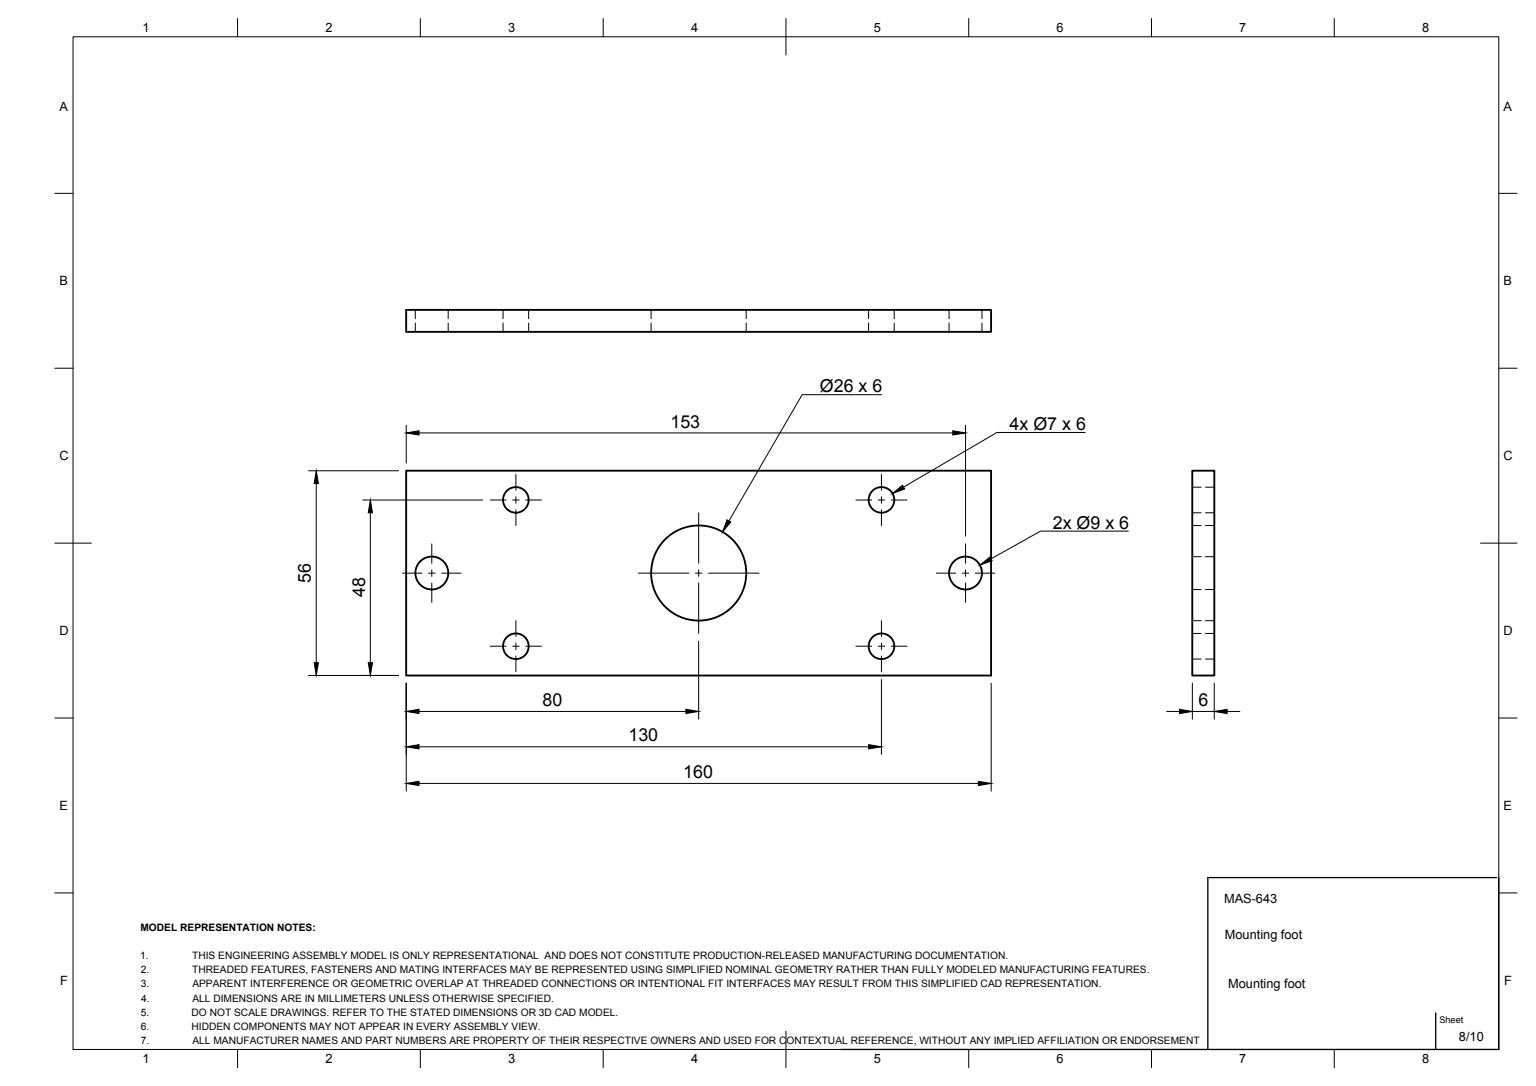
ISO-10303-21;
HEADER;
/* Generated by software containing ST-Developer
 * from STEP Tools, Inc. (www.steptools.com) 
 */

FILE_DESCRIPTION(
/* description */ ('Independent eighteen-tube parallel-flow evaporator geometry. Repeated
 machined headers and gasketed service covers, eighteen copper tubes, 
twenty-nine punched fins, threaded hose connections and bolted mountin
g feet. Native editable features and instanced parts. Braze details, w
orking fluid, pressure and thermal ratings require engineering selecti
on.'),
/* implementation_level */ '2;1');

FILE_NAME(
/* name */ 'Mounting foot.step',
/* time_stamp */ '2026-11-08T20:53:59-08:00',
/* author */ (''),
/* organization */ (''),
/* preprocessor_version */ 'ST-DEVELOPER v20.2',
/* originating_system */ 'Autodesk Translation Framework v15.17.0.0',
/* authorisation */ '');

FILE_SCHEMA (('AUTOMOTIVE_DESIGN { 1 0 10303 214 3 1 1 }'));
ENDSEC;

DATA;
#10=MECHANICAL_DESIGN_GEOMETRIC_PRESENTATION_REPRESENTATION('',(#338),#42620);
#318=SHAPE_REPRESENTATION_RELATIONSHIP('SRR','None',#42728,#328);
#328=ADVANCED_BREP_SHAPE_REPRESENTATION('',(#348),#42615);
#338=STYLED_ITEM('',(#42787),#348);
#348=MANIFOLD_SOLID_BREP('Body1',#10388);
#457=FACE_BOUND('',#1662,.T.);
#458=FACE_BOUND('',#1663,.T.);
#459=FACE_BOUND('',#1664,.T.);
#460=FACE_BOUND('',#1665,.T.);
#461=FACE_BOUND('',#1666,.T.);
#462=FACE_BOUND('',#1667,.T.);
#463=FACE_BOUND('',#1668,.T.);
#464=FACE_BOUND('',#1670,.T.);
#465=FACE_BOUND('',#1671,.T.);
#466=FACE_BOUND('',#1672,.T.);
#467=FACE_BOUND('',#1673,.T.);
#468=FACE_BOUND('',#1674,.T.);
#469=FACE_BOUND('',#1675,.T.);
#470=FACE_BOUND('',#1676,.T.);
#541=PLANE('',#11055);
#542=PLANE('',#11056);
#543=PLANE('',#11057);
#544=PLANE('',#11058);
#545=PLANE('',#11059);
#546=PLANE('',#11060);
#1002=FACE_OUTER_BOUND('',#1650,.T.);
#1003=FACE_OUTER_BOUND('',#1651,.T.);
#1004=FACE_OUTER_BOUND('',#1652,.T.);
#1005=FACE_OUTER_BOUND('',#1653,.T.);
#1006=FACE_OUTER_BOUND('',#1654,.T.);
#1007=FACE_OUTER_BOUND('',#1655,.T.);
#1008=FACE_OUTER_BOUND('',#1656,.T.);
#1009=FACE_OUTER_BOUND('',#1657,.T.);
#1010=FACE_OUTER_BOUND('',#1658,.T.);
#1011=FACE_OUTER_BOUND('',#1659,.T.);
#1012=FACE_OUTER_BOUND('',#1660,.T.);
#1013=FACE_OUTER_BOUND('',#1661,.T.);
#1014=FACE_OUTER_BOUND('',#1669,.T.);
#1650=EDGE_LOOP('',(#8675,#8676,#8677,#8678));
#1651=EDGE_LOOP('',(#8679,#8680,#8681,#8682));
#1652=EDGE_LOOP('',(#8683,#8684,#8685,#8686));
#1653=EDGE_LOOP('',(#8687,#8688,#8689,#8690));
#1654=EDGE_LOOP('',(#8691,#8692,#8693,#8694));
#1655=EDGE_LOOP('',(#8695,#8696,#8697,#8698));
#1656=EDGE_LOOP('',(#8699,#8700,#8701,#8702));
#1657=EDGE_LOOP('',(#8703,#8704,#8705,#8706));
#1658=EDGE_LOOP('',(#8707,#8708,#8709,#8710));
#1659=EDGE_LOOP('',(#8711,#8712,#8713,#8714));
#1660=EDGE_LOOP('',(#8715,#8716,#8717,#8718));
#1661=EDGE_LOOP('',(#8719,#8720,#8721,#8722));
#1662=EDGE_LOOP('',(#8723));
#1663=EDGE_LOOP('',(#8724));
#1664=EDGE_LOOP('',(#8725));
#1665=EDGE_LOOP('',(#8726));
#1666=EDGE_LOOP('',(#8727));
#1667=EDGE_LOOP('',(#8728));
#1668=EDGE_LOOP('',(#8729));
#1669=EDGE_LOOP('',(#8730,#8731,#8732,#8733));
#1670=EDGE_LOOP('',(#8734));
#1671=EDGE_LOOP('',(#8735));
#1672=EDGE_LOOP('',(#8736));
#1673=EDGE_LOOP('',(#8737));
#1674=EDGE_LOOP('',(#8738));
#1675=EDGE_LOOP('',(#8739));
#1676=EDGE_LOOP('',(#8740));
#1967=CIRCLE('',#11035,13.);
#1968=CIRCLE('',#11036,13.);
#1969=CIRCLE('',#11038,4.5);
#1970=CIRCLE('',#11039,4.5);
#1971=CIRCLE('',#11041,4.5);
#1972=CIRCLE('',#11042,4.5);
#1973=CIRCLE('',#11044,3.5);
#1974=CIRCLE('',#11045,3.5);
#1975=CIRCLE('',#11047,3.5);
#1976=CIRCLE('',#11048,3.5);
#1977=CIRCLE('',#11050,3.5);
#1978=CIRCLE('',#11051,3.5);
#1979=CIRCLE('',#11053,3.5);
#1980=CIRCLE('',#11054,3.5);
#3194=LINE('',#35119,#3732);
#3195=LINE('',#35125,#3733);
#3196=LINE('',#35131,#3734);
#3197=LINE('',#35137,#3735);
#3198=LINE('',#35143,#3736);
#3199=LINE('',#35149,#3737);
#3200=LINE('',#35155,#3738);
#3201=LINE('',#35160,#3739);
#3202=LINE('',#35162,#3740);
#3203=LINE('',#35164,#3741);
#3204=LINE('',#35165,#3742);
#3205=LINE('',#35168,#3743);
#3206=LINE('',#35170,#3744);
#3207=LINE('',#35171,#3745);
#3208=LINE('',#35174,#3746);
#3209=LINE('',#35176,#3747);
#3210=LINE('',#35177,#3748);
#3211=LINE('',#35179,#3749);
#3212=LINE('',#35180,#3750);
#3732=VECTOR('',#12765,13.);
#3733=VECTOR('',#12772,4.5);
#3734=VECTOR('',#12779,4.5);
#3735=VECTOR('',#12786,3.5);
#3736=VECTOR('',#12793,3.5);
#3737=VECTOR('',#12800,3.5);
#3738=VECTOR('',#12807,3.5);
#3739=VECTOR('',#12812,10.);
#3740=VECTOR('',#12813,10.);
#3741=VECTOR('',#12814,10.);
#3742=VECTOR('',#12815,10.);
#3743=VECTOR('',#12818,10.);
#3744=VECTOR('',#12819,10.);
#3745=VECTOR('',#12820,10.);
#3746=VECTOR('',#12823,10.);
#3747=VECTOR('',#12824,10.);
#3748=VECTOR('',#12825,10.);
#3749=VECTOR('',#12828,10.);
#3750=VECTOR('',#12829,10.);
#4631=VERTEX_POINT('',#35116);
#4632=VERTEX_POINT('',#35118);
#4633=VERTEX_POINT('',#35122);
#4634=VERTEX_POINT('',#35124);
#4635=VERTEX_POINT('',#35128);
#4636=VERTEX_POINT('',#35130);
#4637=VERTEX_POINT('',#35134);
#4638=VERTEX_POINT('',#35136);
#4639=VERTEX_POINT('',#35140);
#4640=VERTEX_POINT('',#35142);
#4641=VERTEX_POINT('',#35146);
#4642=VERTEX_POINT('',#35148);
#4643=VERTEX_POINT('',#35152);
#4644=VERTEX_POINT('',#35154);
#4645=VERTEX_POINT('',#35158);
#4646=VERTEX_POINT('',#35159);
#4647=VERTEX_POINT('',#35161);
#4648=VERTEX_POINT('',#35163);
#4649=VERTEX_POINT('',#35167);
#4650=VERTEX_POINT('',#35169);
#4651=VERTEX_POINT('',#35173);
#4652=VERTEX_POINT('',#35175);
#6020=EDGE_CURVE('',#4631,#4631,#1967,.T.);
#6021=EDGE_CURVE('',#4631,#4632,#3194,.T.);
#6022=EDGE_CURVE('',#4632,#4632,#1968,.T.);
#6023=EDGE_CURVE('',#4633,#4633,#1969,.T.);
#6024=EDGE_CURVE('',#4633,#4634,#3195,.T.);
#6025=EDGE_CURVE('',#4634,#4634,#1970,.T.);
#6026=EDGE_CURVE('',#4635,#4635,#1971,.T.);
#6027=EDGE_CURVE('',#4635,#4636,#3196,.T.);
#6028=EDGE_CURVE('',#4636,#4636,#1972,.T.);
#6029=EDGE_CURVE('',#4637,#4637,#1973,.T.);
#6030=EDGE_CURVE('',#4637,#4638,#3197,.T.);
#6031=EDGE_CURVE('',#4638,#4638,#1974,.T.);
#6032=EDGE_CURVE('',#4639,#4639,#1975,.T.);
#6033=EDGE_CURVE('',#4639,#4640,#3198,.T.);
#6034=EDGE_CURVE('',#4640,#4640,#1976,.T.);
#6035=EDGE_CURVE('',#4641,#4641,#1977,.T.);
#6036=EDGE_CURVE('',#4641,#4642,#3199,.T.);
#6037=EDGE_CURVE('',#4642,#4642,#1978,.T.);
#6038=EDGE_CURVE('',#4643,#4643,#1979,.T.);
#6039=EDGE_CURVE('',#4643,#4644,#3200,.T.);
#6040=EDGE_CURVE('',#4644,#4644,#1980,.T.);
#6041=EDGE_CURVE('',#4645,#4646,#3201,.T.);
#6042=EDGE_CURVE('',#4646,#4647,#3202,.T.);
#6043=EDGE_CURVE('',#4648,#4647,#3203,.T.);
#6044=EDGE_CURVE('',#4645,#4648,#3204,.T.);
#6045=EDGE_CURVE('',#4649,#4645,#3205,.T.);
#6046=EDGE_CURVE('',#4650,#4648,#3206,.T.);
#6047=EDGE_CURVE('',#4649,#4650,#3207,.T.);
#6048=EDGE_CURVE('',#4651,#4649,#3208,.T.);
#6049=EDGE_CURVE('',#4652,#4650,#3209,.T.);
#6050=EDGE_CURVE('',#4651,#4652,#3210,.T.);
#6051=EDGE_CURVE('',#4646,#4651,#3211,.T.);
#6052=EDGE_CURVE('',#4647,#4652,#3212,.T.);
#8675=ORIENTED_EDGE('',*,*,#6020,.F.);
#8676=ORIENTED_EDGE('',*,*,#6021,.T.);
#8677=ORIENTED_EDGE('',*,*,#6022,.F.);
#8678=ORIENTED_EDGE('',*,*,#6021,.F.);
#8679=ORIENTED_EDGE('',*,*,#6023,.F.);
#8680=ORIENTED_EDGE('',*,*,#6024,.T.);
#8681=ORIENTED_EDGE('',*,*,#6025,.F.);
#8682=ORIENTED_EDGE('',*,*,#6024,.F.);
#8683=ORIENTED_EDGE('',*,*,#6026,.F.);
#8684=ORIENTED_EDGE('',*,*,#6027,.T.);
#8685=ORIENTED_EDGE('',*,*,#6028,.F.);
#8686=ORIENTED_EDGE('',*,*,#6027,.F.);
#8687=ORIENTED_EDGE('',*,*,#6029,.F.);
#8688=ORIENTED_EDGE('',*,*,#6030,.T.);
#8689=ORIENTED_EDGE('',*,*,#6031,.F.);
#8690=ORIENTED_EDGE('',*,*,#6030,.F.);
#8691=ORIENTED_EDGE('',*,*,#6032,.F.);
#8692=ORIENTED_EDGE('',*,*,#6033,.T.);
#8693=ORIENTED_EDGE('',*,*,#6034,.F.);
#8694=ORIENTED_EDGE('',*,*,#6033,.F.);
#8695=ORIENTED_EDGE('',*,*,#6035,.F.);
#8696=ORIENTED_EDGE('',*,*,#6036,.T.);
#8697=ORIENTED_EDGE('',*,*,#6037,.F.);
#8698=ORIENTED_EDGE('',*,*,#6036,.F.);
#8699=ORIENTED_EDGE('',*,*,#6038,.F.);
#8700=ORIENTED_EDGE('',*,*,#6039,.T.);
#8701=ORIENTED_EDGE('',*,*,#6040,.F.);
#8702=ORIENTED_EDGE('',*,*,#6039,.F.);
#8703=ORIENTED_EDGE('',*,*,#6041,.T.);
#8704=ORIENTED_EDGE('',*,*,#6042,.T.);
#8705=ORIENTED_EDGE('',*,*,#6043,.F.);
#8706=ORIENTED_EDGE('',*,*,#6044,.F.);
#8707=ORIENTED_EDGE('',*,*,#6045,.T.);
#8708=ORIENTED_EDGE('',*,*,#6044,.T.);
#8709=ORIENTED_EDGE('',*,*,#6046,.F.);
#8710=ORIENTED_EDGE('',*,*,#6047,.F.);
#8711=ORIENTED_EDGE('',*,*,#6048,.T.);
#8712=ORIENTED_EDGE('',*,*,#6047,.T.);
#8713=ORIENTED_EDGE('',*,*,#6049,.F.);
#8714=ORIENTED_EDGE('',*,*,#6050,.F.);
#8715=ORIENTED_EDGE('',*,*,#6051,.T.);
#8716=ORIENTED_EDGE('',*,*,#6050,.T.);
#8717=ORIENTED_EDGE('',*,*,#6052,.F.);
#8718=ORIENTED_EDGE('',*,*,#6042,.F.);
#8719=ORIENTED_EDGE('',*,*,#6052,.T.);
#8720=ORIENTED_EDGE('',*,*,#6049,.T.);
#8721=ORIENTED_EDGE('',*,*,#6046,.T.);
#8722=ORIENTED_EDGE('',*,*,#6043,.T.);
#8723=ORIENTED_EDGE('',*,*,#6020,.T.);
#8724=ORIENTED_EDGE('',*,*,#6023,.T.);
#8725=ORIENTED_EDGE('',*,*,#6026,.T.);
#8726=ORIENTED_EDGE('',*,*,#6029,.T.);
#8727=ORIENTED_EDGE('',*,*,#6032,.T.);
#8728=ORIENTED_EDGE('',*,*,#6035,.T.);
#8729=ORIENTED_EDGE('',*,*,#6038,.T.);
#8730=ORIENTED_EDGE('',*,*,#6051,.F.);
#8731=ORIENTED_EDGE('',*,*,#6041,.F.);
#8732=ORIENTED_EDGE('',*,*,#6045,.F.);
#8733=ORIENTED_EDGE('',*,*,#6048,.F.);
#8734=ORIENTED_EDGE('',*,*,#6022,.T.);
#8735=ORIENTED_EDGE('',*,*,#6025,.T.);
#8736=ORIENTED_EDGE('',*,*,#6028,.T.);
#8737=ORIENTED_EDGE('',*,*,#6031,.T.);
#8738=ORIENTED_EDGE('',*,*,#6034,.T.);
#8739=ORIENTED_EDGE('',*,*,#6037,.T.);
#8740=ORIENTED_EDGE('',*,*,#6040,.T.);
#9740=CYLINDRICAL_SURFACE('',#11034,13.);
#9741=CYLINDRICAL_SURFACE('',#11037,4.5);
#9742=CYLINDRICAL_SURFACE('',#11040,4.5);
#9743=CYLINDRICAL_SURFACE('',#11043,3.5);
#9744=CYLINDRICAL_SURFACE('',#11046,3.5);
#9745=CYLINDRICAL_SURFACE('',#11049,3.5);
#9746=CYLINDRICAL_SURFACE('',#11052,3.5);
#10238=ADVANCED_FACE('',(#1002),#9740,.F.);
#10239=ADVANCED_FACE('',(#1003),#9741,.F.);
#10240=ADVANCED_FACE('',(#1004),#9742,.F.);
#10241=ADVANCED_FACE('',(#1005),#9743,.F.);
#10242=ADVANCED_FACE('',(#1006),#9744,.F.);
#10243=ADVANCED_FACE('',(#1007),#9745,.F.);
#10244=ADVANCED_FACE('',(#1008),#9746,.F.);
#10245=ADVANCED_FACE('',(#1009),#541,.T.);
#10246=ADVANCED_FACE('',(#1010),#542,.T.);
#10247=ADVANCED_FACE('',(#1011),#543,.T.);
#10248=ADVANCED_FACE('',(#1012),#544,.T.);
#10249=ADVANCED_FACE('',(#1013,#457,#458,#459,#460,#461,#462,#463),#545,
 .T.);
#10250=ADVANCED_FACE('',(#1014,#464,#465,#466,#467,#468,#469,#470),#546,
 .F.);
#10388=CLOSED_SHELL('',(#10238,#10239,#10240,#10241,#10242,#10243,#10244,
#10245,#10246,#10247,#10248,#10249,#10250));
#11033=AXIS2_PLACEMENT_3D('',#35114,#12759,#12760);
#11034=AXIS2_PLACEMENT_3D('',#35115,#12761,#12762);
#11035=AXIS2_PLACEMENT_3D('',#35117,#12763,#12764);
#11036=AXIS2_PLACEMENT_3D('',#35120,#12766,#12767);
#11037=AXIS2_PLACEMENT_3D('',#35121,#12768,#12769);
#11038=AXIS2_PLACEMENT_3D('',#35123,#12770,#12771);
#11039=AXIS2_PLACEMENT_3D('',#35126,#12773,#12774);
#11040=AXIS2_PLACEMENT_3D('',#35127,#12775,#12776);
#11041=AXIS2_PLACEMENT_3D('',#35129,#12777,#12778);
#11042=AXIS2_PLACEMENT_3D('',#35132,#12780,#12781);
#11043=AXIS2_PLACEMENT_3D('',#35133,#12782,#12783);
#11044=AXIS2_PLACEMENT_3D('',#35135,#12784,#12785);
#11045=AXIS2_PLACEMENT_3D('',#35138,#12787,#12788);
#11046=AXIS2_PLACEMENT_3D('',#35139,#12789,#12790);
#11047=AXIS2_PLACEMENT_3D('',#35141,#12791,#12792);
#11048=AXIS2_PLACEMENT_3D('',#35144,#12794,#12795);
#11049=AXIS2_PLACEMENT_3D('',#35145,#12796,#12797);
#11050=AXIS2_PLACEMENT_3D('',#35147,#12798,#12799);
#11051=AXIS2_PLACEMENT_3D('',#35150,#12801,#12802);
#11052=AXIS2_PLACEMENT_3D('',#35151,#12803,#12804);
#11053=AXIS2_PLACEMENT_3D('',#35153,#12805,#12806);
#11054=AXIS2_PLACEMENT_3D('',#35156,#12808,#12809);
#11055=AXIS2_PLACEMENT_3D('',#35157,#12810,#12811);
#11056=AXIS2_PLACEMENT_3D('',#35166,#12816,#12817);
#11057=AXIS2_PLACEMENT_3D('',#35172,#12821,#12822);
#11058=AXIS2_PLACEMENT_3D('',#35178,#12826,#12827);
#11059=AXIS2_PLACEMENT_3D('',#35181,#12830,#12831);
#11060=AXIS2_PLACEMENT_3D('',#35182,#12832,#12833);
#12759=DIRECTION('axis',(0.,0.,1.));
#12760=DIRECTION('refdir',(1.,0.,0.));
#12761=DIRECTION('center_axis',(0.,0.,-1.));
#12762=DIRECTION('ref_axis',(1.,0.,0.));
#12763=DIRECTION('center_axis',(0.,0.,-1.));
#12764=DIRECTION('ref_axis',(1.,0.,0.));
#12765=DIRECTION('',(0.,0.,-1.));
#12766=DIRECTION('center_axis',(0.,0.,1.));
#12767=DIRECTION('ref_axis',(1.,0.,0.));
#12768=DIRECTION('center_axis',(0.,0.,-1.));
#12769=DIRECTION('ref_axis',(1.,0.,0.));
#12770=DIRECTION('center_axis',(0.,0.,-1.));
#12771=DIRECTION('ref_axis',(1.,0.,0.));
#12772=DIRECTION('',(0.,0.,-1.));
#12773=DIRECTION('center_axis',(0.,0.,1.));
#12774=DIRECTION('ref_axis',(1.,0.,0.));
#12775=DIRECTION('center_axis',(0.,0.,-1.));
#12776=DIRECTION('ref_axis',(1.,0.,0.));
#12777=DIRECTION('center_axis',(0.,0.,-1.));
#12778=DIRECTION('ref_axis',(1.,0.,0.));
#12779=DIRECTION('',(0.,0.,-1.));
#12780=DIRECTION('center_axis',(0.,0.,1.));
#12781=DIRECTION('ref_axis',(1.,0.,0.));
#12782=DIRECTION('center_axis',(0.,0.,-1.));
#12783=DIRECTION('ref_axis',(1.,0.,0.));
#12784=DIRECTION('center_axis',(0.,0.,-1.));
#12785=DIRECTION('ref_axis',(1.,0.,0.));
#12786=DIRECTION('',(0.,0.,-1.));
#12787=DIRECTION('center_axis',(0.,0.,1.));
#12788=DIRECTION('ref_axis',(1.,0.,0.));
#12789=DIRECTION('center_axis',(0.,0.,-1.));
#12790=DIRECTION('ref_axis',(1.,0.,0.));
#12791=DIRECTION('center_axis',(0.,0.,-1.));
#12792=DIRECTION('ref_axis',(1.,0.,0.));
#12793=DIRECTION('',(0.,0.,-1.));
#12794=DIRECTION('center_axis',(0.,0.,1.));
#12795=DIRECTION('ref_axis',(1.,0.,0.));
#12796=DIRECTION('center_axis',(0.,0.,-1.));
#12797=DIRECTION('ref_axis',(1.,0.,0.));
#12798=DIRECTION('center_axis',(0.,0.,-1.));
#12799=DIRECTION('ref_axis',(1.,0.,0.));
#12800=DIRECTION('',(0.,0.,-1.));
#12801=DIRECTION('center_axis',(0.,0.,1.));
#12802=DIRECTION('ref_axis',(1.,0.,0.));
#12803=DIRECTION('center_axis',(0.,0.,-1.));
#12804=DIRECTION('ref_axis',(1.,0.,0.));
#12805=DIRECTION('center_axis',(0.,0.,-1.));
#12806=DIRECTION('ref_axis',(1.,0.,0.));
#12807=DIRECTION('',(0.,0.,-1.));
#12808=DIRECTION('center_axis',(0.,0.,1.));
#12809=DIRECTION('ref_axis',(1.,0.,0.));
#12810=DIRECTION('center_axis',(0.,1.,0.));
#12811=DIRECTION('ref_axis',(-1.,0.,0.));
#12812=DIRECTION('',(-1.,0.,0.));
#12813=DIRECTION('',(0.,0.,1.));
#12814=DIRECTION('',(-1.,0.,0.));
#12815=DIRECTION('',(0.,0.,1.));
#12816=DIRECTION('center_axis',(1.,0.,0.));
#12817=DIRECTION('ref_axis',(0.,1.,0.));
#12818=DIRECTION('',(0.,1.,0.));
#12819=DIRECTION('',(0.,1.,0.));
#12820=DIRECTION('',(0.,0.,1.));
#12821=DIRECTION('center_axis',(0.,-1.,0.));
#12822=DIRECTION('ref_axis',(1.,0.,0.));
#12823=DIRECTION('',(1.,0.,0.));
#12824=DIRECTION('',(1.,0.,0.));
#12825=DIRECTION('',(0.,0.,1.));
#12826=DIRECTION('center_axis',(-1.,0.,0.));
#12827=DIRECTION('ref_axis',(0.,-1.,0.));
#12828=DIRECTION('',(0.,-1.,0.));
#12829=DIRECTION('',(0.,-1.,0.));
#12830=DIRECTION('center_axis',(0.,0.,1.));
#12831=DIRECTION('ref_axis',(1.,0.,0.));
#12832=DIRECTION('center_axis',(0.,0.,1.));
#12833=DIRECTION('ref_axis',(1.,0.,0.));
#35114=CARTESIAN_POINT('',(0.,0.,0.));
#35115=CARTESIAN_POINT('Origin',(0.,0.,-43.));
#35116=CARTESIAN_POINT('',(-13.,1.59204083889156E-15,-40.));
#35117=CARTESIAN_POINT('Origin',(0.,0.,-40.));
#35118=CARTESIAN_POINT('',(-13.,1.59204083889156E-15,-46.));
#35119=CARTESIAN_POINT('',(-13.,1.59204083889156E-15,-43.));
#35120=CARTESIAN_POINT('Origin',(0.,0.,-46.));
#35121=CARTESIAN_POINT('Origin',(0.,-73.,-43.));
#35122=CARTESIAN_POINT('',(-4.5,-73.,-40.));
#35123=CARTESIAN_POINT('Origin',(0.,-73.,-40.));
#35124=CARTESIAN_POINT('',(-4.5,-73.,-46.));
#35125=CARTESIAN_POINT('',(-4.5,-73.,-43.));
#35126=CARTESIAN_POINT('Origin',(0.,-73.,-46.));
#35127=CARTESIAN_POINT('Origin',(0.,73.,-43.));
#35128=CARTESIAN_POINT('',(-4.5,73.,-40.));
#35129=CARTESIAN_POINT('Origin',(0.,73.,-40.));
#35130=CARTESIAN_POINT('',(-4.5,73.,-46.));
#35131=CARTESIAN_POINT('',(-4.5,73.,-43.));
#35132=CARTESIAN_POINT('Origin',(0.,73.,-46.));
#35133=CARTESIAN_POINT('Origin',(20.,-50.,-43.));
#35134=CARTESIAN_POINT('',(16.5,-50.,-40.));
#35135=CARTESIAN_POINT('Origin',(20.,-50.,-40.));
#35136=CARTESIAN_POINT('',(16.5,-50.,-46.));
#35137=CARTESIAN_POINT('',(16.5,-50.,-43.));
#35138=CARTESIAN_POINT('Origin',(20.,-50.,-46.));
#35139=CARTESIAN_POINT('Origin',(-20.,-50.,-43.));
#35140=CARTESIAN_POINT('',(-23.5,-50.,-40.));
#35141=CARTESIAN_POINT('Origin',(-20.,-50.,-40.));
#35142=CARTESIAN_POINT('',(-23.5,-50.,-46.));
#35143=CARTESIAN_POINT('',(-23.5,-50.,-43.));
#35144=CARTESIAN_POINT('Origin',(-20.,-50.,-46.));
#35145=CARTESIAN_POINT('Origin',(-20.,50.,-43.));
#35146=CARTESIAN_POINT('',(-23.5,50.,-40.));
#35147=CARTESIAN_POINT('Origin',(-20.,50.,-40.));
#35148=CARTESIAN_POINT('',(-23.5,50.,-46.));
#35149=CARTESIAN_POINT('',(-23.5,50.,-43.));
#35150=CARTESIAN_POINT('Origin',(-20.,50.,-46.));
#35151=CARTESIAN_POINT('Origin',(20.,50.,-43.));
#35152=CARTESIAN_POINT('',(16.5,50.,-40.));
#35153=CARTESIAN_POINT('Origin',(20.,50.,-40.));
#35154=CARTESIAN_POINT('',(16.5,50.,-46.));
#35155=CARTESIAN_POINT('',(16.5,50.,-43.));
#35156=CARTESIAN_POINT('Origin',(20.,50.,-46.));
#35157=CARTESIAN_POINT('Origin',(28.,80.,-46.));
#35158=CARTESIAN_POINT('',(28.,80.,-46.));
#35159=CARTESIAN_POINT('',(-28.,80.,-46.));
#35160=CARTESIAN_POINT('',(28.,80.,-46.));
#35161=CARTESIAN_POINT('',(-28.,80.,-40.));
#35162=CARTESIAN_POINT('',(-28.,80.,-46.));
#35163=CARTESIAN_POINT('',(28.,80.,-40.));
#35164=CARTESIAN_POINT('',(28.,80.,-40.));
#35165=CARTESIAN_POINT('',(28.,80.,-46.));
#35166=CARTESIAN_POINT('Origin',(28.,-80.,-46.));
#35167=CARTESIAN_POINT('',(28.,-80.,-46.));
#35168=CARTESIAN_POINT('',(28.,-80.,-46.));
#35169=CARTESIAN_POINT('',(28.,-80.,-40.));
#35170=CARTESIAN_POINT('',(28.,-80.,-40.));
#35171=CARTESIAN_POINT('',(28.,-80.,-46.));
#35172=CARTESIAN_POINT('Origin',(-28.,-80.,-46.));
#35173=CARTESIAN_POINT('',(-28.,-80.,-46.));
#35174=CARTESIAN_POINT('',(-28.,-80.,-46.));
#35175=CARTESIAN_POINT('',(-28.,-80.,-40.));
#35176=CARTESIAN_POINT('',(-28.,-80.,-40.));
#35177=CARTESIAN_POINT('',(-28.,-80.,-46.));
#35178=CARTESIAN_POINT('Origin',(-28.,80.,-46.));
#35179=CARTESIAN_POINT('',(-28.,80.,-46.));
#35180=CARTESIAN_POINT('',(-28.,80.,-40.));
#35181=CARTESIAN_POINT('Origin',(0.,0.,-40.));
#35182=CARTESIAN_POINT('Origin',(0.,0.,-46.));
#42603=UNCERTAINTY_MEASURE_WITH_UNIT(LENGTH_MEASURE(0.01),#42621,
'DISTANCE_ACCURACY_VALUE',
'Maximum model space distance between geometric entities at asserted c
onnectivities');
#42608=UNCERTAINTY_MEASURE_WITH_UNIT(LENGTH_MEASURE(0.01),#42621,
'DISTANCE_ACCURACY_VALUE',
'Maximum model space distance between geometric entities at asserted c
onnectivities');
#42615=(
GEOMETRIC_REPRESENTATION_CONTEXT(3)
GLOBAL_UNCERTAINTY_ASSIGNED_CONTEXT((#42603))
GLOBAL_UNIT_ASSIGNED_CONTEXT((#42621,#42623,#42624))
REPRESENTATION_CONTEXT('','3D')
);
#42620=(
GEOMETRIC_REPRESENTATION_CONTEXT(3)
GLOBAL_UNCERTAINTY_ASSIGNED_CONTEXT((#42608))
GLOBAL_UNIT_ASSIGNED_CONTEXT((#42621,#42623,#42624))
REPRESENTATION_CONTEXT('','3D')
);
#42621=(
LENGTH_UNIT()
NAMED_UNIT(*)
SI_UNIT(.MILLI.,.METRE.)
);
#42623=(
NAMED_UNIT(*)
PLANE_ANGLE_UNIT()
SI_UNIT($,.RADIAN.)
);
#42624=(
NAMED_UNIT(*)
SI_UNIT($,.STERADIAN.)
SOLID_ANGLE_UNIT()
);
#42631=SHAPE_DEFINITION_REPRESENTATION(#42642,#42728);
#42642=PRODUCT_DEFINITION_SHAPE('',$,#42740);
#42728=SHAPE_REPRESENTATION('',(#11033),#42615);
#42733=PRODUCT_DEFINITION_CONTEXT('part definition',#42768,'design');
#42740=PRODUCT_DEFINITION('Mounting foot','Mounting foot',#42751,#42733);
#42751=PRODUCT_DEFINITION_FORMATION('',$,#42776);
#42768=APPLICATION_CONTEXT(
'Core Data for Automotive Mechanical Design Process');
#42769=PRODUCT_CONTEXT('part definition',#42768,'mechanical');
#42776=PRODUCT('Mounting foot','Mounting foot','Mounting foot',(#42769));
#42787=PRESENTATION_STYLE_ASSIGNMENT((#42795));
#42795=SURFACE_STYLE_USAGE(.BOTH.,#42803);
#42803=SURFACE_SIDE_STYLE('',(#42811));
#42811=SURFACE_STYLE_FILL_AREA(#42819);
#42819=FILL_AREA_STYLE('Gray',(#42827));
#42827=FILL_AREA_STYLE_COLOUR('Gray',#42835);
#42835=COLOUR_RGB('Gray',0.407843137254902,0.447058823529412,0.498039215686275);
ENDSEC;
END-ISO-10303-21;
